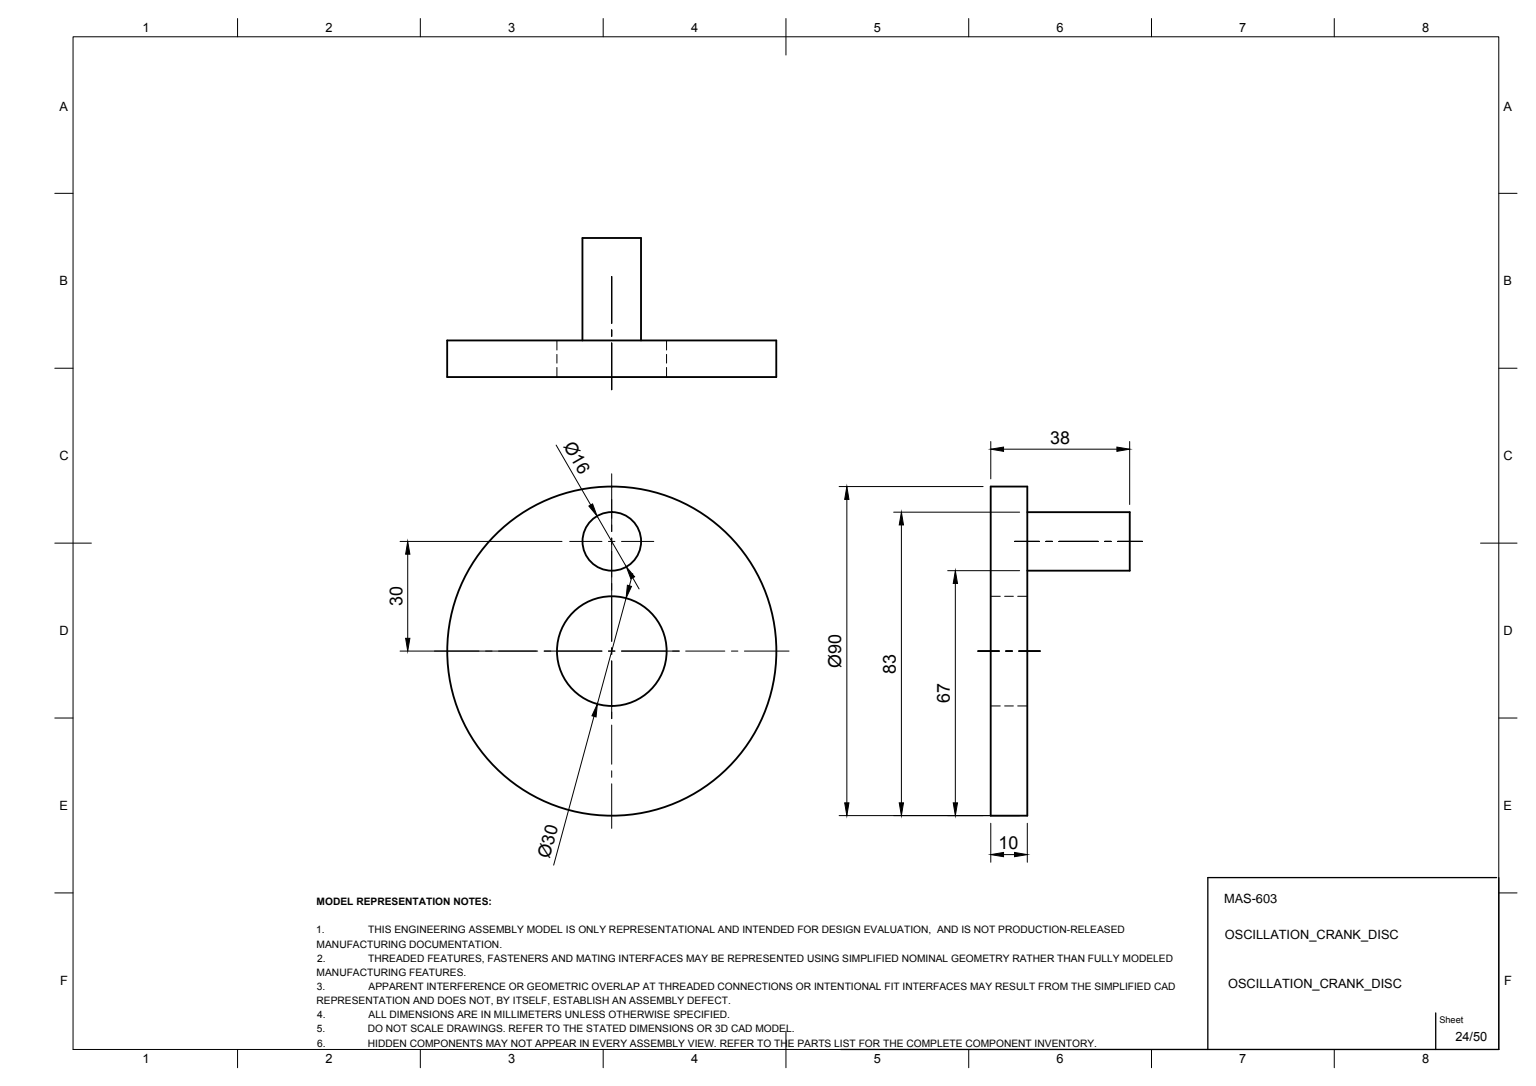
ISO-10303-21;
HEADER;
FILE_DESCRIPTION((''),'2;1');
FILE_NAME('OSCILLATION_CRANK_DISC.step','2026-10-01T22:06:14-07:00',(''),(''),'','','');
FILE_SCHEMA (('AUTOMOTIVE_DESIGN { 1 0 10303 214 3 1 1 }'));
ENDSEC;
DATA;
#10=MECHANICAL_DESIGN_GEOMETRIC_PRESENTATION_REPRESENTATION('',(#996),#50440);
#906=SHAPE_REPRESENTATION_RELATIONSHIP('SRR','None',#50638,#951) ;
#951=ADVANCED_BREP_SHAPE_REPRESENTATION('',(#1051),#50407) ;
#996=STYLED_ITEM('',(#50883),#1051) ;
#1051=MANIFOLD_SOLID_BREP('OSCILLATION_CRANK_DISC',#28663) ;
#1299=FACE_BOUND('',#4927,.T.) ;
#1300=FACE_BOUND('',#4928,.T.) ;
#1301=FACE_BOUND('',#4930,.T.) ;
#2048=PLANE('',#30549) ;
#2049=PLANE('',#30556) ;
#2050=PLANE('',#30557) ;
#3181=FACE_OUTER_BOUND('',#4922,.T.) ;
#3182=FACE_OUTER_BOUND('',#4923,.T.) ;
#3183=FACE_OUTER_BOUND('',#4924,.T.) ;
#3184=FACE_OUTER_BOUND('',#4925,.T.) ;
#3185=FACE_OUTER_BOUND('',#4926,.T.) ;
#3186=FACE_OUTER_BOUND('',#4929,.T.) ;
#4922=EDGE_LOOP('',(#22955,#22956,#22957,#22958)) ;
#4923=EDGE_LOOP('',(#22959)) ;
#4924=EDGE_LOOP('',(#22960,#22961,#22962,#22963)) ;
#4925=EDGE_LOOP('',(#22964,#22965,#22966,#22967)) ;
#4926=EDGE_LOOP('',(#22968)) ;
#4927=EDGE_LOOP('',(#22969)) ;
#4928=EDGE_LOOP('',(#22970)) ;
#4929=EDGE_LOOP('',(#22971)) ;
#4930=EDGE_LOOP('',(#22972)) ;
#7442=LINE('',#45898,#9914) ;
#7443=LINE('',#45905,#9915) ;
#7444=LINE('',#45911,#9916) ;
#9914=VECTOR('',#36763,0.8) ;
#9915=VECTOR('',#36772,1.5) ;
#9916=VECTOR('',#36779,4.5) ;
#11105=CIRCLE('',#30547,0.8) ;
#11106=CIRCLE('',#30548,0.8) ;
#11107=CIRCLE('',#30551,1.5) ;
#11108=CIRCLE('',#30552,1.5) ;
#11109=CIRCLE('',#30554,4.5) ;
#11110=CIRCLE('',#30555,4.5) ;
#13301=VERTEX_POINT('',#45895) ;
#13302=VERTEX_POINT('',#45897) ;
#13303=VERTEX_POINT('',#45902) ;
#13304=VERTEX_POINT('',#45904) ;
#13305=VERTEX_POINT('',#45908) ;
#13306=VERTEX_POINT('',#45910) ;
#16743=EDGE_CURVE('',#13301,#13301,#11105,.T.) ;
#16744=EDGE_CURVE('',#13301,#13302,#7442,.T.) ;
#16745=EDGE_CURVE('',#13302,#13302,#11106,.T.) ;
#16746=EDGE_CURVE('',#13303,#13303,#11107,.T.) ;
#16747=EDGE_CURVE('',#13303,#13304,#7443,.T.) ;
#16748=EDGE_CURVE('',#13304,#13304,#11108,.T.) ;
#16749=EDGE_CURVE('',#13305,#13305,#11109,.T.) ;
#16750=EDGE_CURVE('',#13305,#13306,#7444,.T.) ;
#16751=EDGE_CURVE('',#13306,#13306,#11110,.T.) ;
#22955=ORIENTED_EDGE('',*,*,#16743,.F.) ;
#22956=ORIENTED_EDGE('',*,*,#16744,.T.) ;
#22957=ORIENTED_EDGE('',*,*,#16745,.F.) ;
#22958=ORIENTED_EDGE('',*,*,#16744,.F.) ;
#22959=ORIENTED_EDGE('',*,*,#16745,.T.) ;
#22960=ORIENTED_EDGE('',*,*,#16746,.F.) ;
#22961=ORIENTED_EDGE('',*,*,#16747,.T.) ;
#22962=ORIENTED_EDGE('',*,*,#16748,.F.) ;
#22963=ORIENTED_EDGE('',*,*,#16747,.F.) ;
#22964=ORIENTED_EDGE('',*,*,#16749,.F.) ;
#22965=ORIENTED_EDGE('',*,*,#16750,.T.) ;
#22966=ORIENTED_EDGE('',*,*,#16751,.F.) ;
#22967=ORIENTED_EDGE('',*,*,#16750,.F.) ;
#22968=ORIENTED_EDGE('',*,*,#16751,.T.) ;
#22969=ORIENTED_EDGE('',*,*,#16743,.T.) ;
#22970=ORIENTED_EDGE('',*,*,#16746,.T.) ;
#22971=ORIENTED_EDGE('',*,*,#16749,.T.) ;
#22972=ORIENTED_EDGE('',*,*,#16748,.T.) ;
#26822=CYLINDRICAL_SURFACE('',#30546,0.8) ;
#26823=CYLINDRICAL_SURFACE('',#30550,1.5) ;
#26824=CYLINDRICAL_SURFACE('',#30553,4.5) ;
#27916=ADVANCED_FACE('',(#3181),#26822,.T.) ;
#27917=ADVANCED_FACE('',(#3182),#2048,.T.) ;
#27918=ADVANCED_FACE('',(#3183),#26823,.F.) ;
#27919=ADVANCED_FACE('',(#3184),#26824,.T.) ;
#27920=ADVANCED_FACE('',(#3185,#1299,#1300),#2049,.T.) ;
#27921=ADVANCED_FACE('',(#3186,#1301),#2050,.T.) ;
#28663=CLOSED_SHELL('',(#27916,#27917,#27918,#27919,#27920,#27921)) ;
#30545=AXIS2_PLACEMENT_3D('',#45893,#36757,#36758) ;
#30546=AXIS2_PLACEMENT_3D('',#45894,#36759,#36760) ;
#30547=AXIS2_PLACEMENT_3D('',#45896,#36761,#36762) ;
#30548=AXIS2_PLACEMENT_3D('',#45899,#36764,#36765) ;
#30549=AXIS2_PLACEMENT_3D('',#45900,#36766,#36767) ;
#30550=AXIS2_PLACEMENT_3D('',#45901,#36768,#36769) ;
#30551=AXIS2_PLACEMENT_3D('',#45903,#36770,#36771) ;
#30552=AXIS2_PLACEMENT_3D('',#45906,#36773,#36774) ;
#30553=AXIS2_PLACEMENT_3D('',#45907,#36775,#36776) ;
#30554=AXIS2_PLACEMENT_3D('',#45909,#36777,#36778) ;
#30555=AXIS2_PLACEMENT_3D('',#45912,#36780,#36781) ;
#30556=AXIS2_PLACEMENT_3D('',#45913,#36782,#36783) ;
#30557=AXIS2_PLACEMENT_3D('',#45914,#36784,#36785) ;
#36757=DIRECTION('axis',(0.,0.,1.)) ;
#36758=DIRECTION('refdir',(1.,0.,0.)) ;
#36759=DIRECTION('center_axis',(0.,1.,0.)) ;
#36760=DIRECTION('ref_axis',(1.,0.,0.)) ;
#36761=DIRECTION('center_axis',(0.,1.,0.)) ;
#36762=DIRECTION('ref_axis',(1.,0.,0.)) ;
#36763=DIRECTION('',(0.,-1.,0.)) ;
#36764=DIRECTION('center_axis',(0.,-1.,0.)) ;
#36765=DIRECTION('ref_axis',(1.,0.,0.)) ;
#36766=DIRECTION('center_axis',(0.,-1.,0.)) ;
#36767=DIRECTION('ref_axis',(-1.,0.,0.)) ;
#36768=DIRECTION('center_axis',(0.,1.,0.)) ;
#36769=DIRECTION('ref_axis',(1.,0.,0.)) ;
#36770=DIRECTION('center_axis',(0.,1.,0.)) ;
#36771=DIRECTION('ref_axis',(1.,0.,0.)) ;
#36772=DIRECTION('',(0.,1.,0.)) ;
#36773=DIRECTION('center_axis',(0.,-1.,0.)) ;
#36774=DIRECTION('ref_axis',(1.,0.,0.)) ;
#36775=DIRECTION('center_axis',(0.,1.,0.)) ;
#36776=DIRECTION('ref_axis',(1.,0.,0.)) ;
#36777=DIRECTION('center_axis',(0.,1.,0.)) ;
#36778=DIRECTION('ref_axis',(1.,0.,0.)) ;
#36779=DIRECTION('',(0.,-1.,0.)) ;
#36780=DIRECTION('center_axis',(0.,-1.,0.)) ;
#36781=DIRECTION('ref_axis',(1.,0.,0.)) ;
#36782=DIRECTION('center_axis',(0.,-1.,0.)) ;
#36783=DIRECTION('ref_axis',(-1.,0.,0.)) ;
#36784=DIRECTION('center_axis',(0.,1.,0.)) ;
#36785=DIRECTION('ref_axis',(1.,0.,0.)) ;
#45893=CARTESIAN_POINT('',(0.,0.,0.)) ;
#45894=CARTESIAN_POINT('Origin',(3.,-15.4,37.)) ;
#45895=CARTESIAN_POINT('',(2.2,-14.,37.)) ;
#45896=CARTESIAN_POINT('Origin',(3.,-14.,37.)) ;
#45897=CARTESIAN_POINT('',(2.2,-16.8,37.)) ;
#45898=CARTESIAN_POINT('',(2.2,-15.4,37.)) ;
#45899=CARTESIAN_POINT('Origin',(3.,-16.8,37.)) ;
#45900=CARTESIAN_POINT('Origin',(3.,-16.8,37.)) ;
#45901=CARTESIAN_POINT('Origin',(0.,-13.5,37.)) ;
#45902=CARTESIAN_POINT('',(-1.5,-14.,37.)) ;
#45903=CARTESIAN_POINT('Origin',(0.,-14.,37.)) ;
#45904=CARTESIAN_POINT('',(-1.5,-13.,37.)) ;
#45905=CARTESIAN_POINT('',(-1.5,-13.5,37.)) ;
#45906=CARTESIAN_POINT('Origin',(0.,-13.,37.)) ;
#45907=CARTESIAN_POINT('Origin',(0.,-13.5,37.)) ;
#45908=CARTESIAN_POINT('',(-4.5,-13.,37.)) ;
#45909=CARTESIAN_POINT('Origin',(0.,-13.,37.)) ;
#45910=CARTESIAN_POINT('',(-4.5,-14.,37.)) ;
#45911=CARTESIAN_POINT('',(-4.5,-13.5,37.)) ;
#45912=CARTESIAN_POINT('Origin',(0.,-14.,37.)) ;
#45913=CARTESIAN_POINT('Origin',(0.,-14.,37.)) ;
#45914=CARTESIAN_POINT('Origin',(0.,-13.,37.)) ;
#50354=UNCERTAINTY_MEASURE_WITH_UNIT(LENGTH_MEASURE(0.001),#50441,
'DISTANCE_ACCURACY_VALUE',
'Maximum model space distance between geometric entities at asserted c
onnectivities') ;
#50387=UNCERTAINTY_MEASURE_WITH_UNIT(LENGTH_MEASURE(0.001),#50441,
'DISTANCE_ACCURACY_VALUE',
'Maximum model space distance between geometric entities at asserted c
onnectivities') ;
#50407=(
GEOMETRIC_REPRESENTATION_CONTEXT(3)
GLOBAL_UNCERTAINTY_ASSIGNED_CONTEXT((#50354))
GLOBAL_UNIT_ASSIGNED_CONTEXT((#50441,#50443,#50444))
REPRESENTATION_CONTEXT('','3D')
) ;
#50440=(
GEOMETRIC_REPRESENTATION_CONTEXT(3)
GLOBAL_UNCERTAINTY_ASSIGNED_CONTEXT((#50387))
GLOBAL_UNIT_ASSIGNED_CONTEXT((#50441,#50443,#50444))
REPRESENTATION_CONTEXT('','3D')
) ;
#50441=(
LENGTH_UNIT()
NAMED_UNIT(*)
SI_UNIT(.CENTI.,.METRE.)
) ;
#50443=(
NAMED_UNIT(*)
PLANE_ANGLE_UNIT()
SI_UNIT($,.RADIAN.)
) ;
#50444=(
NAMED_UNIT(*)
SI_UNIT($,.STERADIAN.)
SOLID_ANGLE_UNIT()
) ;
#50464=SHAPE_DEFINITION_REPRESENTATION(#50530,#50638) ;
#50530=PRODUCT_DEFINITION_SHAPE('',$,#50691) ;
#50638=SHAPE_REPRESENTATION('',(#30545),#50407) ;
#50671=PRODUCT_DEFINITION_CONTEXT('part definition',#50829,'design') ;
#50691=PRODUCT_DEFINITION('OSCILLATION_CRANK_DISC',
'OSCILLATION_CRANK_DISC',#50743,#50671) ;
#50743=PRODUCT_DEFINITION_FORMATION('',$,#50850) ;
#50829=APPLICATION_CONTEXT(
'Core Data for Automotive Mechanical Design Process') ;
#50830=PRODUCT_CONTEXT('part definition',#50829,'mechanical') ;
#50850=PRODUCT('OSCILLATION_CRANK_DISC','OSCILLATION_CRANK_DISC',$,(#50830)) ;
#50883=PRESENTATION_STYLE_ASSIGNMENT((#50890)) ;
#50890=SURFACE_STYLE_USAGE(.BOTH.,#50897) ;
#50897=SURFACE_SIDE_STYLE('',(#50904)) ;
#50904=SURFACE_STYLE_FILL_AREA(#50911) ;
#50911=FILL_AREA_STYLE('Steel - Satin',(#50918)) ;
#50918=FILL_AREA_STYLE_COLOUR('Steel - Satin',#50925) ;
#50925=COLOUR_RGB('Steel - Satin', 0.31764706, 0.68627451, 0.89019608) ;
ENDSEC;
END-ISO-10303-21;
